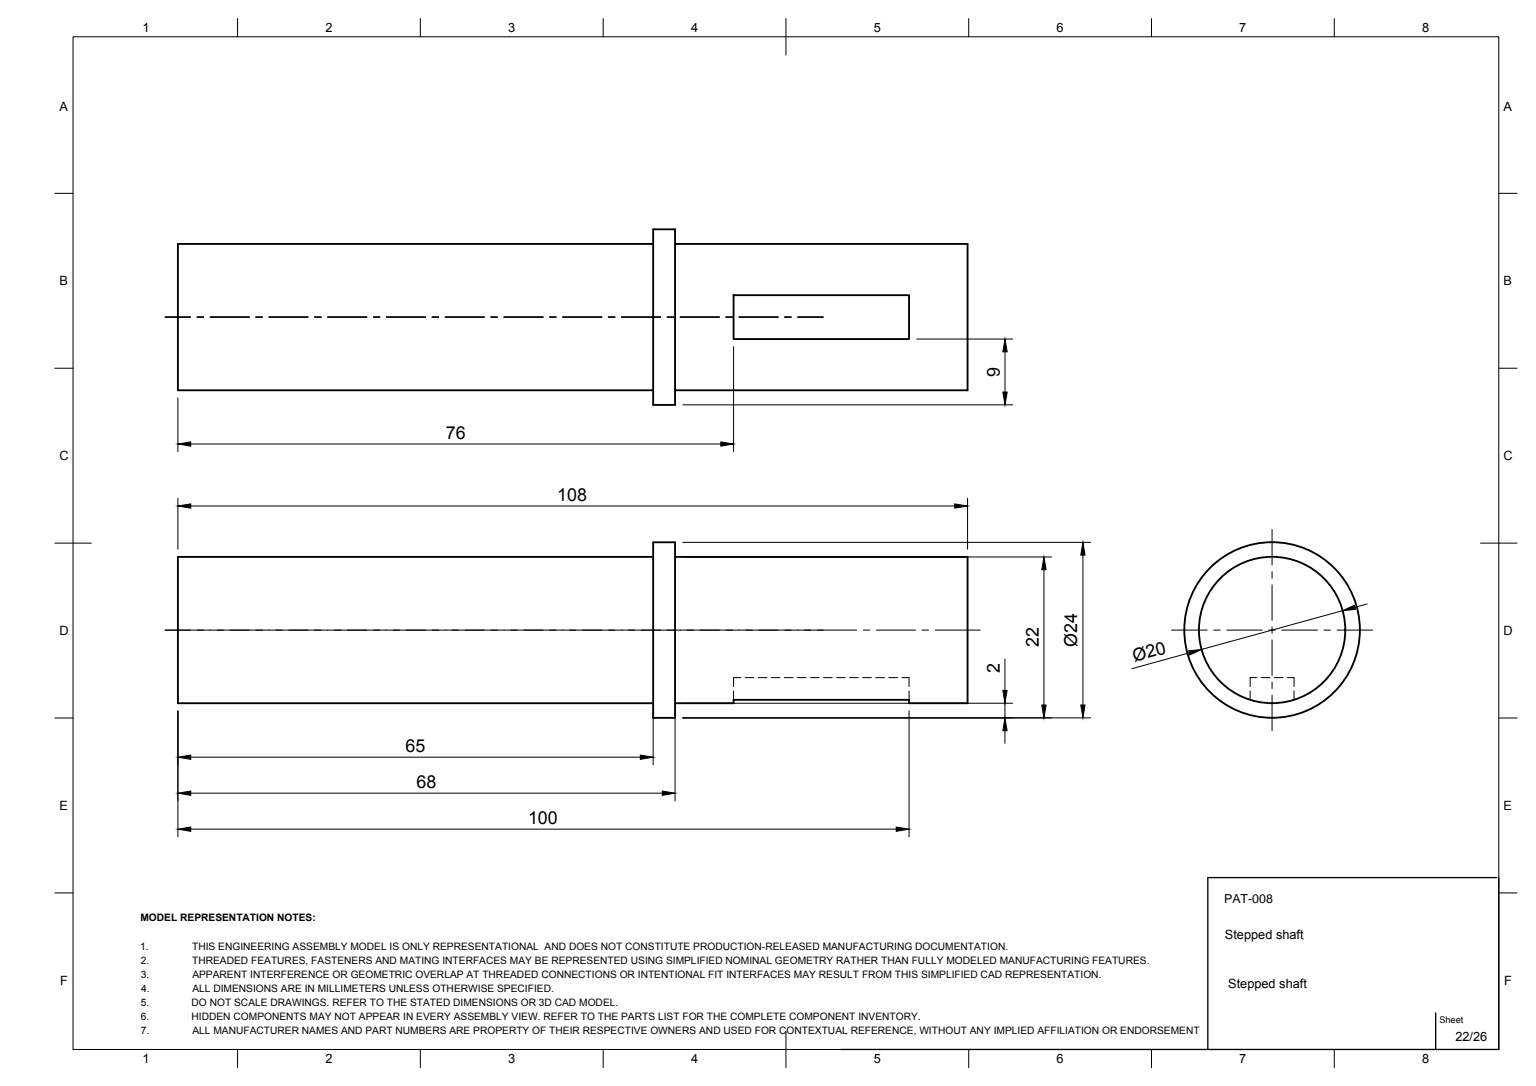
ISO-10303-21;
HEADER;
/* Generated by software containing ST-Developer
 * from STEP Tools, Inc. (www.steptools.com) 
 */

FILE_DESCRIPTION(
/* description */ ('Bearing housing with oil seal and end cap'),
/* implementation_level */ '2;1');

FILE_NAME(
/* name */ 'Stepped shaft.step',
/* time_stamp */ '2026-10-28T03:23:10-07:00',
/* author */ (''),
/* organization */ (''),
/* preprocessor_version */ 'ST-DEVELOPER v20.2',
/* originating_system */ 'Autodesk Translation Framework v15.17.0.0',
/* authorisation */ '');

FILE_SCHEMA (('AUTOMOTIVE_DESIGN { 1 0 10303 214 3 1 1 }'));
ENDSEC;

DATA;
#10=MECHANICAL_DESIGN_GEOMETRIC_PRESENTATION_REPRESENTATION('',(#282),#7871);
#232=SHAPE_REPRESENTATION_RELATIONSHIP('SRR','None',#7981,#253);
#253=ADVANCED_BREP_SHAPE_REPRESENTATION('',(#309),#7865);
#282=STYLED_ITEM('',(#8153),#309);
#309=MANIFOLD_SOLID_BREP('Body1',#4110);
#385=FACE_BOUND('',#1069,.T.);
#386=FACE_BOUND('',#1071,.T.);
#387=FACE_BOUND('',#1074,.T.);
#510=PLANE('',#4765);
#511=PLANE('',#4766);
#512=PLANE('',#4768);
#513=PLANE('',#4769);
#514=PLANE('',#4770);
#515=PLANE('',#4772);
#516=PLANE('',#4775);
#517=PLANE('',#4783);
#518=PLANE('',#4784);
#742=FACE_OUTER_BOUND('',#1063,.T.);
#743=FACE_OUTER_BOUND('',#1064,.T.);
#744=FACE_OUTER_BOUND('',#1065,.T.);
#745=FACE_OUTER_BOUND('',#1066,.T.);
#746=FACE_OUTER_BOUND('',#1067,.T.);
#747=FACE_OUTER_BOUND('',#1068,.T.);
#748=FACE_OUTER_BOUND('',#1070,.T.);
#749=FACE_OUTER_BOUND('',#1072,.T.);
#750=FACE_OUTER_BOUND('',#1073,.T.);
#751=FACE_OUTER_BOUND('',#1075,.T.);
#752=FACE_OUTER_BOUND('',#1076,.T.);
#753=FACE_OUTER_BOUND('',#1077,.T.);
#1063=EDGE_LOOP('',(#3495,#3496,#3497,#3498));
#1064=EDGE_LOOP('',(#3499,#3500,#3501,#3502));
#1065=EDGE_LOOP('',(#3503,#3504,#3505,#3506));
#1066=EDGE_LOOP('',(#3507,#3508,#3509,#3510));
#1067=EDGE_LOOP('',(#3511,#3512,#3513,#3514));
#1068=EDGE_LOOP('',(#3515));
#1069=EDGE_LOOP('',(#3516));
#1070=EDGE_LOOP('',(#3517));
#1071=EDGE_LOOP('',(#3518));
#1072=EDGE_LOOP('',(#3519,#3520,#3521,#3522));
#1073=EDGE_LOOP('',(#3523,#3524,#3525,#3526));
#1074=EDGE_LOOP('',(#3527,#3528,#3529,#3530));
#1075=EDGE_LOOP('',(#3531,#3532,#3533,#3534));
#1076=EDGE_LOOP('',(#3535));
#1077=EDGE_LOOP('',(#3536));
#1325=LINE('',#7416,#1587);
#1326=LINE('',#7418,#1588);
#1327=LINE('',#7420,#1589);
#1328=LINE('',#7421,#1590);
#1329=LINE('',#7426,#1591);
#1330=LINE('',#7427,#1592);
#1331=LINE('',#7430,#1593);
#1332=LINE('',#7432,#1594);
#1333=LINE('',#7433,#1595);
#1334=LINE('',#7435,#1596);
#1335=LINE('',#7449,#1597);
#1336=LINE('',#7452,#1598);
#1337=LINE('',#7457,#1599);
#1587=VECTOR('',#5894,1.);
#1588=VECTOR('',#5895,1.);
#1589=VECTOR('',#5896,1.);
#1590=VECTOR('',#5897,1.);
#1591=VECTOR('',#5902,1.);
#1592=VECTOR('',#5903,1.);
#1593=VECTOR('',#5906,1.);
#1594=VECTOR('',#5907,1.);
#1595=VECTOR('',#5908,1.);
#1596=VECTOR('',#5911,1.);
#1597=VECTOR('',#5930,1.2);
#1598=VECTOR('',#5933,1.);
#1599=VECTOR('',#5940,1.);
#1851=CIRCLE('',#4767,1.);
#1852=CIRCLE('',#4771,1.);
#1853=CIRCLE('',#4773,1.2);
#1854=CIRCLE('',#4774,1.);
#1855=CIRCLE('',#4776,1.2);
#1856=CIRCLE('',#4777,1.);
#1857=CIRCLE('',#4780,1.);
#1858=CIRCLE('',#4782,1.);
#2147=VERTEX_POINT('',#7414);
#2148=VERTEX_POINT('',#7415);
#2149=VERTEX_POINT('',#7417);
#2150=VERTEX_POINT('',#7419);
#2151=VERTEX_POINT('',#7423);
#2152=VERTEX_POINT('',#7425);
#2153=VERTEX_POINT('',#7429);
#2154=VERTEX_POINT('',#7431);
#2155=VERTEX_POINT('',#7439);
#2156=VERTEX_POINT('',#7441);
#2157=VERTEX_POINT('',#7444);
#2158=VERTEX_POINT('',#7446);
#2159=VERTEX_POINT('',#7451);
#2160=VERTEX_POINT('',#7455);
#2611=EDGE_CURVE('',#2147,#2148,#1325,.T.);
#2612=EDGE_CURVE('',#2147,#2149,#1326,.T.);
#2613=EDGE_CURVE('',#2150,#2149,#1327,.T.);
#2614=EDGE_CURVE('',#2150,#2148,#1328,.T.);
#2615=EDGE_CURVE('',#2148,#2151,#1851,.T.);
#2616=EDGE_CURVE('',#2152,#2150,#1329,.T.);
#2617=EDGE_CURVE('',#2151,#2152,#1330,.T.);
#2618=EDGE_CURVE('',#2151,#2153,#1331,.T.);
#2619=EDGE_CURVE('',#2152,#2154,#1332,.T.);
#2620=EDGE_CURVE('',#2154,#2153,#1333,.T.);
#2621=EDGE_CURVE('',#2149,#2154,#1334,.T.);
#2622=EDGE_CURVE('',#2153,#2147,#1852,.T.);
#2623=EDGE_CURVE('',#2155,#2155,#1853,.T.);
#2624=EDGE_CURVE('',#2156,#2156,#1854,.T.);
#2625=EDGE_CURVE('',#2157,#2157,#1855,.T.);
#2626=EDGE_CURVE('',#2158,#2158,#1856,.T.);
#2627=EDGE_CURVE('',#2155,#2157,#1335,.T.);
#2628=EDGE_CURVE('',#2158,#2159,#1336,.T.);
#2629=EDGE_CURVE('',#2159,#2159,#1857,.T.);
#2630=EDGE_CURVE('',#2160,#2160,#1858,.T.);
#2631=EDGE_CURVE('',#2160,#2156,#1337,.T.);
#3495=ORIENTED_EDGE('',*,*,#2611,.F.);
#3496=ORIENTED_EDGE('',*,*,#2612,.T.);
#3497=ORIENTED_EDGE('',*,*,#2613,.F.);
#3498=ORIENTED_EDGE('',*,*,#2614,.T.);
#3499=ORIENTED_EDGE('',*,*,#2615,.F.);
#3500=ORIENTED_EDGE('',*,*,#2614,.F.);
#3501=ORIENTED_EDGE('',*,*,#2616,.F.);
#3502=ORIENTED_EDGE('',*,*,#2617,.F.);
#3503=ORIENTED_EDGE('',*,*,#2618,.F.);
#3504=ORIENTED_EDGE('',*,*,#2617,.T.);
#3505=ORIENTED_EDGE('',*,*,#2619,.T.);
#3506=ORIENTED_EDGE('',*,*,#2620,.T.);
#3507=ORIENTED_EDGE('',*,*,#2616,.T.);
#3508=ORIENTED_EDGE('',*,*,#2613,.T.);
#3509=ORIENTED_EDGE('',*,*,#2621,.T.);
#3510=ORIENTED_EDGE('',*,*,#2619,.F.);
#3511=ORIENTED_EDGE('',*,*,#2622,.F.);
#3512=ORIENTED_EDGE('',*,*,#2620,.F.);
#3513=ORIENTED_EDGE('',*,*,#2621,.F.);
#3514=ORIENTED_EDGE('',*,*,#2612,.F.);
#3515=ORIENTED_EDGE('',*,*,#2623,.T.);
#3516=ORIENTED_EDGE('',*,*,#2624,.F.);
#3517=ORIENTED_EDGE('',*,*,#2625,.F.);
#3518=ORIENTED_EDGE('',*,*,#2626,.F.);
#3519=ORIENTED_EDGE('',*,*,#2623,.F.);
#3520=ORIENTED_EDGE('',*,*,#2627,.T.);
#3521=ORIENTED_EDGE('',*,*,#2625,.T.);
#3522=ORIENTED_EDGE('',*,*,#2627,.F.);
#3523=ORIENTED_EDGE('',*,*,#2626,.T.);
#3524=ORIENTED_EDGE('',*,*,#2628,.T.);
#3525=ORIENTED_EDGE('',*,*,#2629,.T.);
#3526=ORIENTED_EDGE('',*,*,#2628,.F.);
#3527=ORIENTED_EDGE('',*,*,#2618,.T.);
#3528=ORIENTED_EDGE('',*,*,#2622,.T.);
#3529=ORIENTED_EDGE('',*,*,#2611,.T.);
#3530=ORIENTED_EDGE('',*,*,#2615,.T.);
#3531=ORIENTED_EDGE('',*,*,#2630,.F.);
#3532=ORIENTED_EDGE('',*,*,#2631,.T.);
#3533=ORIENTED_EDGE('',*,*,#2624,.T.);
#3534=ORIENTED_EDGE('',*,*,#2631,.F.);
#3535=ORIENTED_EDGE('',*,*,#2630,.T.);
#3536=ORIENTED_EDGE('',*,*,#2629,.F.);
#3817=CYLINDRICAL_SURFACE('',#4778,1.2);
#3818=CYLINDRICAL_SURFACE('',#4779,1.);
#3819=CYLINDRICAL_SURFACE('',#4781,1.);
#4024=ADVANCED_FACE('',(#742),#510,.F.);
#4025=ADVANCED_FACE('',(#743),#511,.T.);
#4026=ADVANCED_FACE('',(#744),#512,.F.);
#4027=ADVANCED_FACE('',(#745),#513,.F.);
#4028=ADVANCED_FACE('',(#746),#514,.F.);
#4029=ADVANCED_FACE('',(#747,#385),#515,.T.);
#4030=ADVANCED_FACE('',(#748,#386),#516,.F.);
#4031=ADVANCED_FACE('',(#749),#3817,.T.);
#4032=ADVANCED_FACE('',(#750,#387),#3818,.T.);
#4033=ADVANCED_FACE('',(#751),#3819,.T.);
#4034=ADVANCED_FACE('',(#752),#517,.T.);
#4035=ADVANCED_FACE('',(#753),#518,.F.);
#4110=CLOSED_SHELL('',(#4024,#4025,#4026,#4027,#4028,#4029,#4030,#4031,
#4032,#4033,#4034,#4035));
#4764=AXIS2_PLACEMENT_3D('',#7412,#5890,#5891);
#4765=AXIS2_PLACEMENT_3D('',#7413,#5892,#5893);
#4766=AXIS2_PLACEMENT_3D('',#7422,#5898,#5899);
#4767=AXIS2_PLACEMENT_3D('',#7424,#5900,#5901);
#4768=AXIS2_PLACEMENT_3D('',#7428,#5904,#5905);
#4769=AXIS2_PLACEMENT_3D('',#7434,#5909,#5910);
#4770=AXIS2_PLACEMENT_3D('',#7436,#5912,#5913);
#4771=AXIS2_PLACEMENT_3D('',#7437,#5914,#5915);
#4772=AXIS2_PLACEMENT_3D('',#7438,#5916,#5917);
#4773=AXIS2_PLACEMENT_3D('',#7440,#5918,#5919);
#4774=AXIS2_PLACEMENT_3D('',#7442,#5920,#5921);
#4775=AXIS2_PLACEMENT_3D('',#7443,#5922,#5923);
#4776=AXIS2_PLACEMENT_3D('',#7445,#5924,#5925);
#4777=AXIS2_PLACEMENT_3D('',#7447,#5926,#5927);
#4778=AXIS2_PLACEMENT_3D('',#7448,#5928,#5929);
#4779=AXIS2_PLACEMENT_3D('',#7450,#5931,#5932);
#4780=AXIS2_PLACEMENT_3D('',#7453,#5934,#5935);
#4781=AXIS2_PLACEMENT_3D('',#7454,#5936,#5937);
#4782=AXIS2_PLACEMENT_3D('',#7456,#5938,#5939);
#4783=AXIS2_PLACEMENT_3D('',#7458,#5941,#5942);
#4784=AXIS2_PLACEMENT_3D('',#7459,#5943,#5944);
#5890=DIRECTION('axis',(0.,0.,1.));
#5891=DIRECTION('refdir',(1.,0.,0.));
#5892=DIRECTION('center_axis',(-1.,0.,0.));
#5893=DIRECTION('ref_axis',(0.,0.,1.));
#5894=DIRECTION('',(0.,-1.,0.));
#5895=DIRECTION('',(0.,0.,1.));
#5896=DIRECTION('',(0.,1.,0.));
#5897=DIRECTION('',(0.,0.,-1.));
#5898=DIRECTION('center_axis',(0.,1.,0.));
#5899=DIRECTION('ref_axis',(1.,0.,0.));
#5900=DIRECTION('center_axis',(0.,-1.,0.));
#5901=DIRECTION('ref_axis',(1.,0.,0.));
#5902=DIRECTION('',(-1.,0.,0.));
#5903=DIRECTION('',(0.,0.,1.));
#5904=DIRECTION('center_axis',(1.,0.,0.));
#5905=DIRECTION('ref_axis',(0.,0.,-1.));
#5906=DIRECTION('',(0.,1.,0.));
#5907=DIRECTION('',(0.,1.,0.));
#5908=DIRECTION('',(0.,0.,-1.));
#5909=DIRECTION('center_axis',(0.,0.,1.));
#5910=DIRECTION('ref_axis',(1.,0.,0.));
#5911=DIRECTION('',(1.,0.,0.));
#5912=DIRECTION('center_axis',(0.,1.,0.));
#5913=DIRECTION('ref_axis',(0.,0.,1.));
#5914=DIRECTION('center_axis',(0.,1.,0.));
#5915=DIRECTION('ref_axis',(1.,0.,0.));
#5916=DIRECTION('center_axis',(0.,1.,0.));
#5917=DIRECTION('ref_axis',(1.,0.,0.));
#5918=DIRECTION('center_axis',(0.,1.,0.));
#5919=DIRECTION('ref_axis',(1.,0.,0.));
#5920=DIRECTION('center_axis',(0.,1.,0.));
#5921=DIRECTION('ref_axis',(1.,0.,0.));
#5922=DIRECTION('center_axis',(0.,1.,0.));
#5923=DIRECTION('ref_axis',(1.,0.,0.));
#5924=DIRECTION('center_axis',(0.,1.,0.));
#5925=DIRECTION('ref_axis',(1.,0.,0.));
#5926=DIRECTION('center_axis',(0.,-1.,0.));
#5927=DIRECTION('ref_axis',(1.,0.,0.));
#5928=DIRECTION('center_axis',(0.,1.,0.));
#5929=DIRECTION('ref_axis',(1.,0.,0.));
#5930=DIRECTION('',(0.,-1.,0.));
#5931=DIRECTION('center_axis',(0.,1.,0.));
#5932=DIRECTION('ref_axis',(1.,0.,0.));
#5933=DIRECTION('',(0.,-1.,0.));
#5934=DIRECTION('center_axis',(0.,1.,0.));
#5935=DIRECTION('ref_axis',(1.,0.,0.));
#5936=DIRECTION('center_axis',(0.,1.,0.));
#5937=DIRECTION('ref_axis',(1.,0.,0.));
#5938=DIRECTION('center_axis',(0.,1.,0.));
#5939=DIRECTION('ref_axis',(1.,0.,0.));
#5940=DIRECTION('',(0.,-1.,0.));
#5941=DIRECTION('center_axis',(0.,1.,0.));
#5942=DIRECTION('ref_axis',(1.,0.,0.));
#5943=DIRECTION('center_axis',(0.,1.,0.));
#5944=DIRECTION('ref_axis',(1.,0.,0.));
#7412=CARTESIAN_POINT('',(0.,0.,0.));
#7413=CARTESIAN_POINT('Origin',(-0.3,-3.2,3.4));
#7414=CARTESIAN_POINT('',(-0.3,-0.8,3.54606079858305));
#7415=CARTESIAN_POINT('',(-0.3,-3.2,3.54606079858305));
#7416=CARTESIAN_POINT('',(-0.3,-4.,3.54606079858305));
#7417=CARTESIAN_POINT('',(-0.3,-0.8,3.85));
#7418=CARTESIAN_POINT('',(-0.3,-0.8,3.85));
#7419=CARTESIAN_POINT('',(-0.3,-3.2,3.85));
#7420=CARTESIAN_POINT('',(-0.3,-3.2,3.85));
#7421=CARTESIAN_POINT('',(-0.3,-3.2,3.85));
#7422=CARTESIAN_POINT('Origin',(0.,-3.2,3.625));
#7423=CARTESIAN_POINT('',(0.3,-3.2,3.54606079858305));
#7424=CARTESIAN_POINT('Origin',(0.,-3.2,4.5));
#7425=CARTESIAN_POINT('',(0.3,-3.2,3.85));
#7426=CARTESIAN_POINT('',(0.3,-3.2,3.85));
#7427=CARTESIAN_POINT('',(0.3,-3.2,3.4));
#7428=CARTESIAN_POINT('Origin',(0.3,-3.2,3.85));
#7429=CARTESIAN_POINT('',(0.3,-0.8,3.54606079858305));
#7430=CARTESIAN_POINT('',(0.3,-4.,3.54606079858305));
#7431=CARTESIAN_POINT('',(0.3,-0.8,3.85));
#7432=CARTESIAN_POINT('',(0.3,-3.2,3.85));
#7433=CARTESIAN_POINT('',(0.3,-0.8,3.4));
#7434=CARTESIAN_POINT('Origin',(-0.3,-3.2,3.85));
#7435=CARTESIAN_POINT('',(0.3,-0.8,3.85));
#7436=CARTESIAN_POINT('Origin',(0.,-0.8,3.625));
#7437=CARTESIAN_POINT('Origin',(0.,-0.8,4.5));
#7438=CARTESIAN_POINT('Origin',(0.,0.3,4.5));
#7439=CARTESIAN_POINT('',(-1.2,0.3,4.5));
#7440=CARTESIAN_POINT('Origin',(0.,0.3,4.5));
#7441=CARTESIAN_POINT('',(-1.,0.3,4.5));
#7442=CARTESIAN_POINT('Origin',(0.,0.3,4.5));
#7443=CARTESIAN_POINT('Origin',(0.,0.,4.5));
#7444=CARTESIAN_POINT('',(-1.2,0.,4.5));
#7445=CARTESIAN_POINT('Origin',(0.,0.,4.5));
#7446=CARTESIAN_POINT('',(-1.,0.,4.5));
#7447=CARTESIAN_POINT('Origin',(0.,0.,4.5));
#7448=CARTESIAN_POINT('Origin',(0.,0.,4.5));
#7449=CARTESIAN_POINT('',(-1.2,0.,4.5));
#7450=CARTESIAN_POINT('Origin',(0.,-4.,4.5));
#7451=CARTESIAN_POINT('',(-1.,-4.,4.5));
#7452=CARTESIAN_POINT('',(-1.,-4.,4.5));
#7453=CARTESIAN_POINT('Origin',(0.,-4.,4.5));
#7454=CARTESIAN_POINT('Origin',(0.,-4.,4.5));
#7455=CARTESIAN_POINT('',(-1.,6.8,4.5));
#7456=CARTESIAN_POINT('Origin',(0.,6.8,4.5));
#7457=CARTESIAN_POINT('',(-1.,-4.,4.5));
#7458=CARTESIAN_POINT('Origin',(0.,6.8,4.5));
#7459=CARTESIAN_POINT('Origin',(0.,-4.,4.5));
#7839=UNCERTAINTY_MEASURE_WITH_UNIT(LENGTH_MEASURE(0.001),#7872,
'DISTANCE_ACCURACY_VALUE',
'Maximum model space distance between geometric entities at asserted c
onnectivities');
#7845=UNCERTAINTY_MEASURE_WITH_UNIT(LENGTH_MEASURE(0.001),#7872,
'DISTANCE_ACCURACY_VALUE',
'Maximum model space distance between geometric entities at asserted c
onnectivities');
#7865=(
GEOMETRIC_REPRESENTATION_CONTEXT(3)
GLOBAL_UNCERTAINTY_ASSIGNED_CONTEXT((#7839))
GLOBAL_UNIT_ASSIGNED_CONTEXT((#7872,#7874,#7875))
REPRESENTATION_CONTEXT('','3D')
);
#7871=(
GEOMETRIC_REPRESENTATION_CONTEXT(3)
GLOBAL_UNCERTAINTY_ASSIGNED_CONTEXT((#7845))
GLOBAL_UNIT_ASSIGNED_CONTEXT((#7872,#7874,#7875))
REPRESENTATION_CONTEXT('','3D')
);
#7872=(
LENGTH_UNIT()
NAMED_UNIT(*)
SI_UNIT(.CENTI.,.METRE.)
);
#7874=(
NAMED_UNIT(*)
PLANE_ANGLE_UNIT()
SI_UNIT($,.RADIAN.)
);
#7875=(
NAMED_UNIT(*)
SI_UNIT($,.STERADIAN.)
SOLID_ANGLE_UNIT()
);
#7895=SHAPE_DEFINITION_REPRESENTATION(#7947,#7981);
#7947=PRODUCT_DEFINITION_SHAPE('',$,#8007);
#7981=SHAPE_REPRESENTATION('',(#4764),#7865);
#7987=PRODUCT_DEFINITION_CONTEXT('part definition',#8064,'design');
#8007=PRODUCT_DEFINITION('Stepped shaft','Stepped shaft',#8032,#7987);
#8032=PRODUCT_DEFINITION_FORMATION('',$,#8085);
#8064=APPLICATION_CONTEXT(
'Core Data for Automotive Mechanical Design Process');
#8065=PRODUCT_CONTEXT('part definition',#8064,'mechanical');
#8085=PRODUCT('Stepped shaft','Stepped shaft','Stepped shaft',(#8065));
#8147=COLOUR_RGB('Grey',0.48,0.52,0.57);
#8148=FILL_AREA_STYLE_COLOUR('',#8147);
#8149=FILL_AREA_STYLE('',(#8148));
#8150=SURFACE_STYLE_FILL_AREA(#8149);
#8151=SURFACE_SIDE_STYLE('',(#8150));
#8152=SURFACE_STYLE_USAGE(.BOTH.,#8151);
#8153=PRESENTATION_STYLE_ASSIGNMENT((#8152));
ENDSEC;
END-ISO-10303-21;
